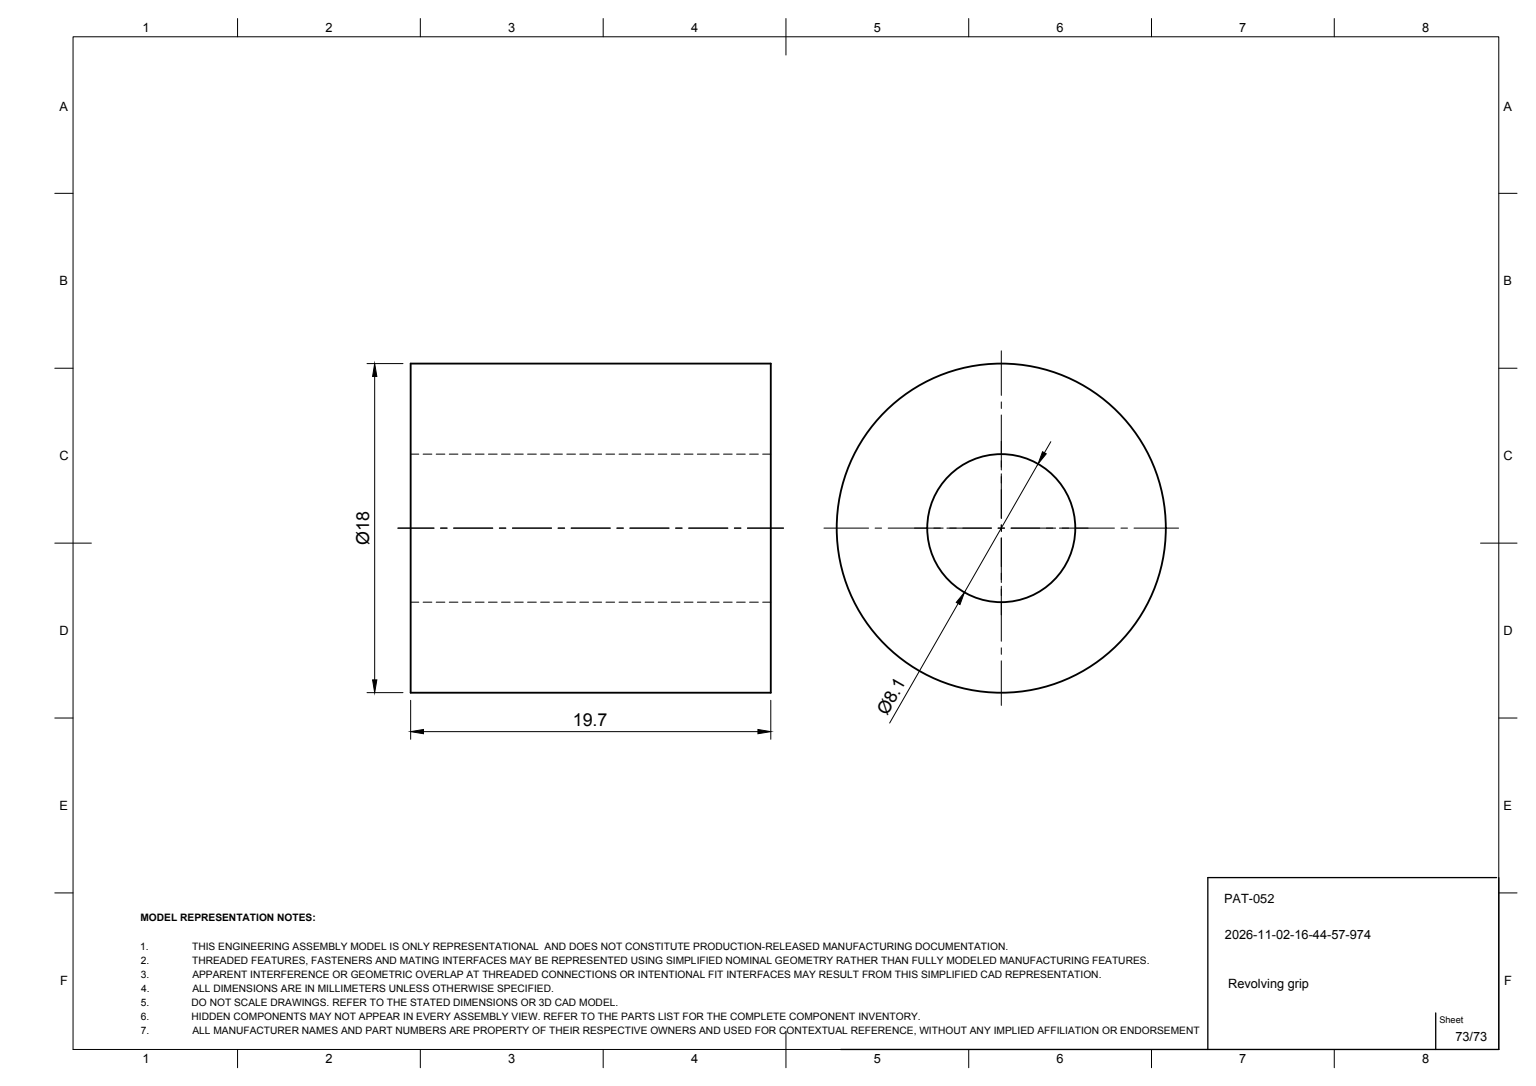
ISO-10303-21;
HEADER;
/* Generated by software containing ST-Developer
 * from STEP Tools, Inc. (www.steptools.com) 
 */

FILE_DESCRIPTION(
/* description */ ('Hand-crank gear train demonstrator'),
/* implementation_level */ '2;1');

FILE_NAME(
/* name */ 'Revolving grip.step',
/* time_stamp */ '2026-10-28T03:22:13-07:00',
/* author */ (''),
/* organization */ (''),
/* preprocessor_version */ 'ST-DEVELOPER v20.2',
/* originating_system */ 'Autodesk Translation Framework v15.17.0.0',
/* authorisation */ '');

FILE_SCHEMA (('AUTOMOTIVE_DESIGN { 1 0 10303 214 3 1 1 }'));
ENDSEC;

DATA;
#10=MECHANICAL_DESIGN_GEOMETRIC_PRESENTATION_REPRESENTATION('',(#1267),#62758);
#1124=SHAPE_REPRESENTATION_RELATIONSHIP('SRR','None',#63103,#1188);
#1188=ADVANCED_BREP_SHAPE_REPRESENTATION('',(#1341),#62757);
#1267=STYLED_ITEM('',(#63469),#1341);
#1341=MANIFOLD_SOLID_BREP('Body1',#16452);
#1631=FACE_BOUND('',#4283,.T.);
#1632=FACE_BOUND('',#4285,.T.);
#2121=PLANE('',#18822);
#2122=PLANE('',#18823);
#3055=FACE_OUTER_BOUND('',#4280,.T.);
#3056=FACE_OUTER_BOUND('',#4281,.T.);
#3057=FACE_OUTER_BOUND('',#4282,.T.);
#3058=FACE_OUTER_BOUND('',#4284,.T.);
#4280=EDGE_LOOP('',(#15155,#15156,#15157,#15158));
#4281=EDGE_LOOP('',(#15159,#15160,#15161,#15162));
#4282=EDGE_LOOP('',(#15163));
#4283=EDGE_LOOP('',(#15164));
#4284=EDGE_LOOP('',(#15165));
#4285=EDGE_LOOP('',(#15166));
#5416=LINE('',#62594,#6548);
#5417=LINE('',#62600,#6549);
#6548=VECTOR('',#23281,0.405);
#6549=VECTOR('',#23288,0.9);
#7208=CIRCLE('',#18817,0.405);
#7209=CIRCLE('',#18818,0.405);
#7210=CIRCLE('',#18820,0.9);
#7211=CIRCLE('',#18821,0.9);
#8665=VERTEX_POINT('',#62591);
#8666=VERTEX_POINT('',#62593);
#8667=VERTEX_POINT('',#62597);
#8668=VERTEX_POINT('',#62599);
#10829=EDGE_CURVE('',#8665,#8665,#7208,.T.);
#10830=EDGE_CURVE('',#8665,#8666,#5416,.T.);
#10831=EDGE_CURVE('',#8666,#8666,#7209,.T.);
#10832=EDGE_CURVE('',#8667,#8667,#7210,.T.);
#10833=EDGE_CURVE('',#8667,#8668,#5417,.T.);
#10834=EDGE_CURVE('',#8668,#8668,#7211,.T.);
#15155=ORIENTED_EDGE('',*,*,#10829,.F.);
#15156=ORIENTED_EDGE('',*,*,#10830,.T.);
#15157=ORIENTED_EDGE('',*,*,#10831,.T.);
#15158=ORIENTED_EDGE('',*,*,#10830,.F.);
#15159=ORIENTED_EDGE('',*,*,#10832,.F.);
#15160=ORIENTED_EDGE('',*,*,#10833,.T.);
#15161=ORIENTED_EDGE('',*,*,#10834,.T.);
#15162=ORIENTED_EDGE('',*,*,#10833,.F.);
#15163=ORIENTED_EDGE('',*,*,#10832,.T.);
#15164=ORIENTED_EDGE('',*,*,#10829,.T.);
#15165=ORIENTED_EDGE('',*,*,#10834,.F.);
#15166=ORIENTED_EDGE('',*,*,#10831,.F.);
#15431=CYLINDRICAL_SURFACE('',#18816,0.405);
#15432=CYLINDRICAL_SURFACE('',#18819,0.9);
#16365=ADVANCED_FACE('',(#3055),#15431,.F.);
#16366=ADVANCED_FACE('',(#3056),#15432,.T.);
#16367=ADVANCED_FACE('',(#3057,#1631),#2121,.T.);
#16368=ADVANCED_FACE('',(#3058,#1632),#2122,.F.);
#16452=CLOSED_SHELL('',(#16365,#16366,#16367,#16368));
#18815=AXIS2_PLACEMENT_3D('',#62589,#23275,#23276);
#18816=AXIS2_PLACEMENT_3D('',#62590,#23277,#23278);
#18817=AXIS2_PLACEMENT_3D('',#62592,#23279,#23280);
#18818=AXIS2_PLACEMENT_3D('',#62595,#23282,#23283);
#18819=AXIS2_PLACEMENT_3D('',#62596,#23284,#23285);
#18820=AXIS2_PLACEMENT_3D('',#62598,#23286,#23287);
#18821=AXIS2_PLACEMENT_3D('',#62601,#23289,#23290);
#18822=AXIS2_PLACEMENT_3D('',#62602,#23291,#23292);
#18823=AXIS2_PLACEMENT_3D('',#62603,#23293,#23294);
#23275=DIRECTION('axis',(0.,0.,1.));
#23276=DIRECTION('refdir',(1.,0.,0.));
#23277=DIRECTION('center_axis',(0.,1.,0.));
#23278=DIRECTION('ref_axis',(1.,0.,0.));
#23279=DIRECTION('center_axis',(0.,-1.,0.));
#23280=DIRECTION('ref_axis',(1.,0.,0.));
#23281=DIRECTION('',(0.,-1.,0.));
#23282=DIRECTION('center_axis',(0.,-1.,0.));
#23283=DIRECTION('ref_axis',(1.,0.,0.));
#23284=DIRECTION('center_axis',(0.,1.,0.));
#23285=DIRECTION('ref_axis',(1.,0.,0.));
#23286=DIRECTION('center_axis',(0.,1.,0.));
#23287=DIRECTION('ref_axis',(1.,0.,0.));
#23288=DIRECTION('',(0.,-1.,0.));
#23289=DIRECTION('center_axis',(0.,1.,0.));
#23290=DIRECTION('ref_axis',(1.,0.,0.));
#23291=DIRECTION('center_axis',(0.,1.,0.));
#23292=DIRECTION('ref_axis',(1.,0.,0.));
#23293=DIRECTION('center_axis',(0.,1.,0.));
#23294=DIRECTION('ref_axis',(1.,0.,0.));
#62589=CARTESIAN_POINT('',(0.,0.,0.));
#62590=CARTESIAN_POINT('Origin',(0.,4.8,13.));
#62591=CARTESIAN_POINT('',(-0.405,6.77,13.));
#62592=CARTESIAN_POINT('Origin',(0.,6.77,13.));
#62593=CARTESIAN_POINT('',(-0.405,4.8,13.));
#62594=CARTESIAN_POINT('',(-0.405,4.8,13.));
#62595=CARTESIAN_POINT('Origin',(0.,4.8,13.));
#62596=CARTESIAN_POINT('Origin',(0.,4.8,13.));
#62597=CARTESIAN_POINT('',(-0.9,6.77,13.));
#62598=CARTESIAN_POINT('Origin',(0.,6.77,13.));
#62599=CARTESIAN_POINT('',(-0.9,4.8,13.));
#62600=CARTESIAN_POINT('',(-0.9,4.8,13.));
#62601=CARTESIAN_POINT('Origin',(0.,4.8,13.));
#62602=CARTESIAN_POINT('Origin',(0.,6.77,13.));
#62603=CARTESIAN_POINT('Origin',(0.,4.8,13.));
#62683=UNCERTAINTY_MEASURE_WITH_UNIT(LENGTH_MEASURE(0.001),#62759,
'DISTANCE_ACCURACY_VALUE',
'Maximum model space distance between geometric entities at asserted c
onnectivities');
#62684=UNCERTAINTY_MEASURE_WITH_UNIT(LENGTH_MEASURE(0.001),#62759,
'DISTANCE_ACCURACY_VALUE',
'Maximum model space distance between geometric entities at asserted c
onnectivities');
#62757=(
GEOMETRIC_REPRESENTATION_CONTEXT(3)
GLOBAL_UNCERTAINTY_ASSIGNED_CONTEXT((#62683))
GLOBAL_UNIT_ASSIGNED_CONTEXT((#62759,#62761,#62762))
REPRESENTATION_CONTEXT('','3D')
);
#62758=(
GEOMETRIC_REPRESENTATION_CONTEXT(3)
GLOBAL_UNCERTAINTY_ASSIGNED_CONTEXT((#62684))
GLOBAL_UNIT_ASSIGNED_CONTEXT((#62759,#62761,#62762))
REPRESENTATION_CONTEXT('','3D')
);
#62759=(
LENGTH_UNIT()
NAMED_UNIT(*)
SI_UNIT(.CENTI.,.METRE.)
);
#62761=(
NAMED_UNIT(*)
PLANE_ANGLE_UNIT()
SI_UNIT($,.RADIAN.)
);
#62762=(
NAMED_UNIT(*)
SI_UNIT($,.STERADIAN.)
SOLID_ANGLE_UNIT()
);
#62835=SHAPE_DEFINITION_REPRESENTATION(#63023,#63103);
#63023=PRODUCT_DEFINITION_SHAPE('',$,#63177);
#63103=SHAPE_REPRESENTATION('',(#18815),#62757);
#63104=PRODUCT_DEFINITION_CONTEXT('part definition',#63325,'design');
#63177=PRODUCT_DEFINITION('Revolving grip','Revolving grip',#63250,#63104);
#63250=PRODUCT_DEFINITION_FORMATION('',$,#63399);
#63325=APPLICATION_CONTEXT(
'Core Data for Automotive Mechanical Design Process');
#63326=PRODUCT_CONTEXT('part definition',#63325,'mechanical');
#63399=PRODUCT('Revolving grip','Revolving grip','Revolving grip',(#63326));
#63463=COLOUR_RGB('Black',0.12,0.14,0.17);
#63464=FILL_AREA_STYLE_COLOUR('',#63463);
#63465=FILL_AREA_STYLE('',(#63464));
#63466=SURFACE_STYLE_FILL_AREA(#63465);
#63467=SURFACE_SIDE_STYLE('',(#63466));
#63468=SURFACE_STYLE_USAGE(.BOTH.,#63467);
#63469=PRESENTATION_STYLE_ASSIGNMENT((#63468));
ENDSEC;
END-ISO-10303-21;
